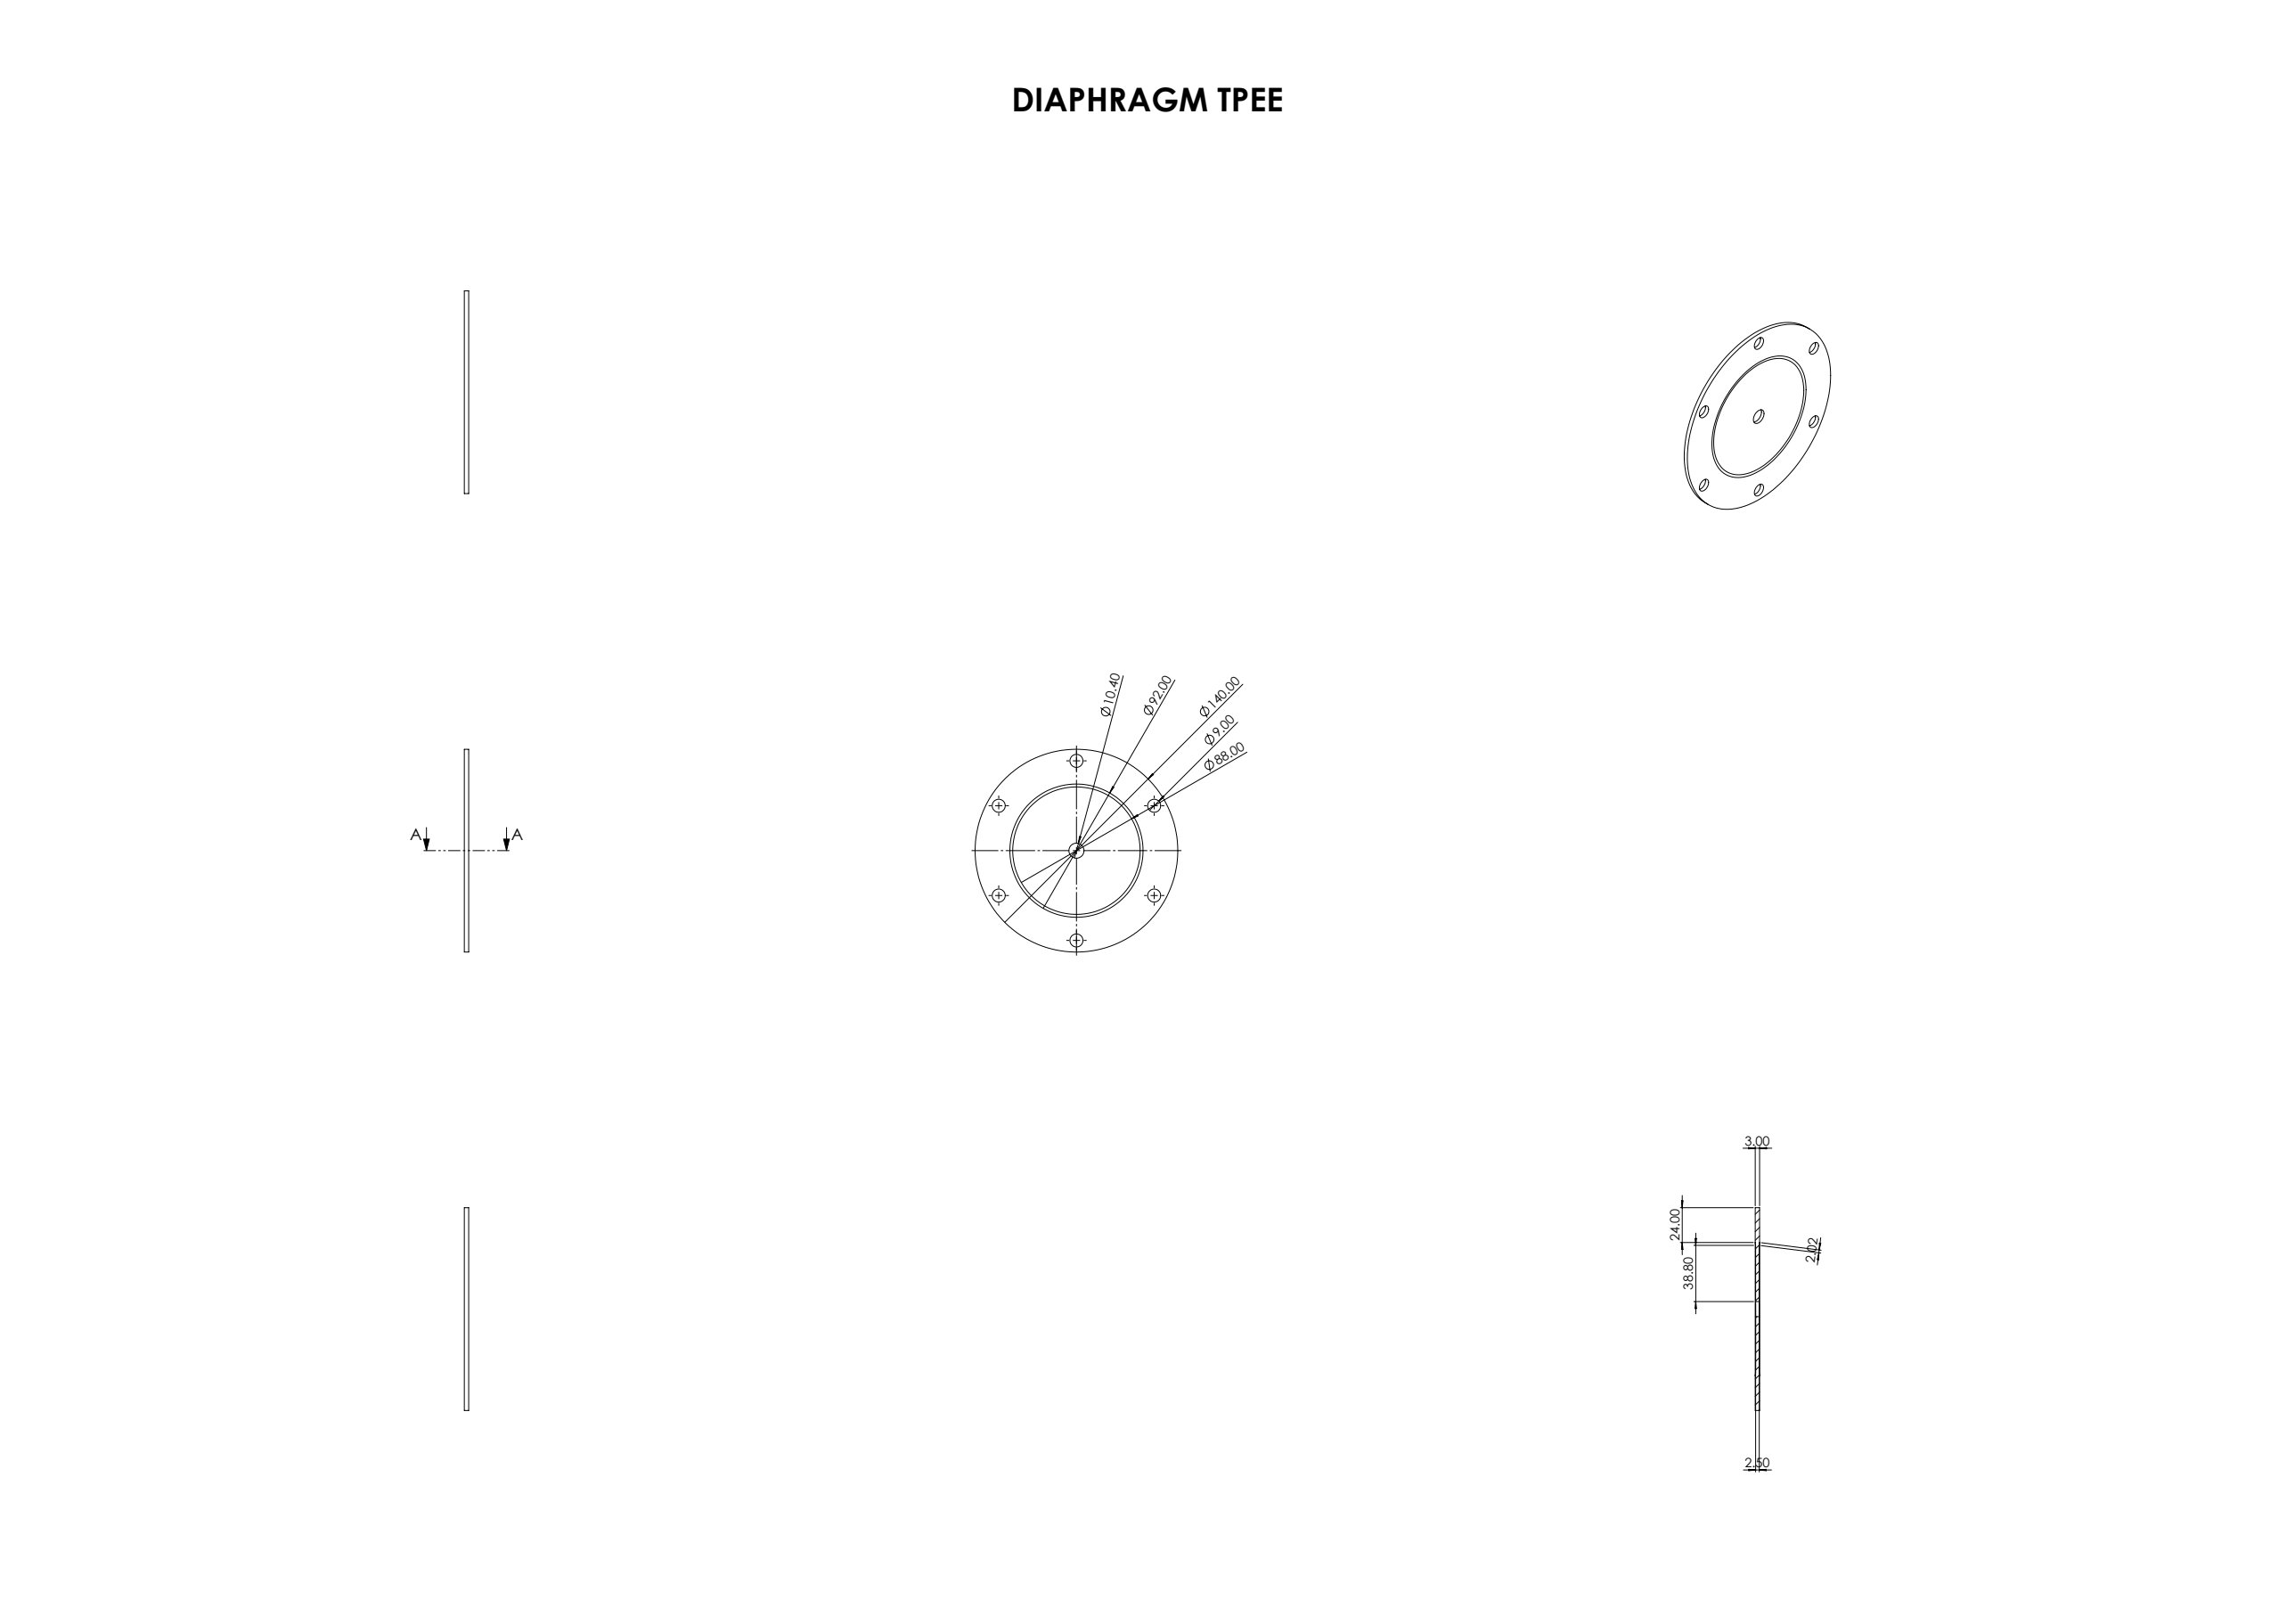
ISO-10303-21;
HEADER;
/* Generated by software containing ST-Developer
 * from STEP Tools, Inc. (www.steptools.com) 
 */

FILE_DESCRIPTION(
/* description */ (''),
/* implementation_level */ '2;1');

FILE_NAME(
/* name */ '05_Diaphragm_TPEE.step',
/* time_stamp */ '2026-10-26T06:13:19-07:00',
/* author */ (''),
/* organization */ (''),
/* preprocessor_version */ 'ST-DEVELOPER v20.2',
/* originating_system */ 'Autodesk Translation Framework v15.15.0.0',
/* authorisation */ '');

FILE_SCHEMA (('AUTOMOTIVE_DESIGN { 1 0 10303 214 3 1 1 }','TECHNICAL_DATA_PACKAGING'));
ENDSEC;

DATA;
#10=MECHANICAL_DESIGN_GEOMETRIC_PRESENTATION_REPRESENTATION('',(#301),#56639);
#261=SHAPE_REPRESENTATION_RELATIONSHIP('SRR','None',#56749,#281);
#281=ADVANCED_BREP_SHAPE_REPRESENTATION('',(#321),#56623);
#301=STYLED_ITEM('',(#56901),#321);
#321=MANIFOLD_SOLID_BREP('Body1',#16953);
#490=FACE_BOUND('',#3058,.T.);
#491=FACE_BOUND('',#3061,.T.);
#492=FACE_BOUND('',#3062,.T.);
#493=FACE_BOUND('',#3063,.T.);
#494=FACE_BOUND('',#3064,.T.);
#495=FACE_BOUND('',#3065,.T.);
#496=FACE_BOUND('',#3066,.T.);
#497=FACE_BOUND('',#3067,.T.);
#498=FACE_BOUND('',#3070,.T.);
#499=FACE_BOUND('',#3071,.T.);
#500=FACE_BOUND('',#3072,.T.);
#501=FACE_BOUND('',#3073,.T.);
#502=FACE_BOUND('',#3074,.T.);
#503=FACE_BOUND('',#3075,.T.);
#504=FACE_BOUND('',#3076,.T.);
#505=FACE_BOUND('',#3079,.T.);
#587=CONICAL_SURFACE('',#17639,45.,1.44644133224813);
#588=CONICAL_SURFACE('',#17647,45.,1.44644133224814);
#888=CIRCLE('',#17617,4.5);
#889=CIRCLE('',#17618,4.5);
#890=CIRCLE('',#17620,4.5);
#891=CIRCLE('',#17621,4.5);
#892=CIRCLE('',#17623,4.5);
#893=CIRCLE('',#17624,4.5);
#894=CIRCLE('',#17626,4.5);
#895=CIRCLE('',#17627,4.5);
#896=CIRCLE('',#17629,4.5);
#897=CIRCLE('',#17630,4.5);
#898=CIRCLE('',#17632,4.5);
#899=CIRCLE('',#17633,4.5);
#900=CIRCLE('',#17635,5.2);
#901=CIRCLE('',#17636,5.2);
#902=CIRCLE('',#17638,44.);
#903=CIRCLE('',#17640,46.);
#904=CIRCLE('',#17642,70.);
#905=CIRCLE('',#17644,70.);
#906=CIRCLE('',#17646,46.);
#907=CIRCLE('',#17648,44.);
#1309=CYLINDRICAL_SURFACE('',#17616,4.5);
#1310=CYLINDRICAL_SURFACE('',#17619,4.5);
#1311=CYLINDRICAL_SURFACE('',#17622,4.5);
#1312=CYLINDRICAL_SURFACE('',#17625,4.5);
#1313=CYLINDRICAL_SURFACE('',#17628,4.5);
#1314=CYLINDRICAL_SURFACE('',#17631,4.5);
#1315=CYLINDRICAL_SURFACE('',#17634,5.2);
#1316=CYLINDRICAL_SURFACE('',#17643,70.);
#2001=FACE_OUTER_BOUND('',#3050,.T.);
#2002=FACE_OUTER_BOUND('',#3051,.T.);
#2003=FACE_OUTER_BOUND('',#3052,.T.);
#2004=FACE_OUTER_BOUND('',#3053,.T.);
#2005=FACE_OUTER_BOUND('',#3054,.T.);
#2006=FACE_OUTER_BOUND('',#3055,.T.);
#2007=FACE_OUTER_BOUND('',#3056,.T.);
#2008=FACE_OUTER_BOUND('',#3057,.T.);
#2009=FACE_OUTER_BOUND('',#3059,.T.);
#2010=FACE_OUTER_BOUND('',#3060,.T.);
#2011=FACE_OUTER_BOUND('',#3068,.T.);
#2012=FACE_OUTER_BOUND('',#3069,.T.);
#2013=FACE_OUTER_BOUND('',#3077,.T.);
#2014=FACE_OUTER_BOUND('',#3078,.T.);
#3050=EDGE_LOOP('',(#11732,#11733,#11734,#11735));
#3051=EDGE_LOOP('',(#11736,#11737,#11738,#11739));
#3052=EDGE_LOOP('',(#11740,#11741,#11742,#11743));
#3053=EDGE_LOOP('',(#11744,#11745,#11746,#11747));
#3054=EDGE_LOOP('',(#11748,#11749,#11750,#11751));
#3055=EDGE_LOOP('',(#11752,#11753,#11754,#11755));
#3056=EDGE_LOOP('',(#11756,#11757,#11758,#11759));
#3057=EDGE_LOOP('',(#11760));
#3058=EDGE_LOOP('',(#11761));
#3059=EDGE_LOOP('',(#11762,#11763,#11764,#11765));
#3060=EDGE_LOOP('',(#11766));
#3061=EDGE_LOOP('',(#11767));
#3062=EDGE_LOOP('',(#11768));
#3063=EDGE_LOOP('',(#11769));
#3064=EDGE_LOOP('',(#11770));
#3065=EDGE_LOOP('',(#11771));
#3066=EDGE_LOOP('',(#11772));
#3067=EDGE_LOOP('',(#11773));
#3068=EDGE_LOOP('',(#11774,#11775,#11776,#11777));
#3069=EDGE_LOOP('',(#11778));
#3070=EDGE_LOOP('',(#11779));
#3071=EDGE_LOOP('',(#11780));
#3072=EDGE_LOOP('',(#11781));
#3073=EDGE_LOOP('',(#11782));
#3074=EDGE_LOOP('',(#11783));
#3075=EDGE_LOOP('',(#11784));
#3076=EDGE_LOOP('',(#11785));
#3077=EDGE_LOOP('',(#11786,#11787,#11788,#11789));
#3078=EDGE_LOOP('',(#11790));
#3079=EDGE_LOOP('',(#11791));
#4083=LINE('',#24999,#5037);
#4084=LINE('',#25005,#5038);
#4085=LINE('',#25011,#5039);
#4086=LINE('',#25017,#5040);
#4087=LINE('',#25023,#5041);
#4088=LINE('',#25029,#5042);
#4089=LINE('',#25035,#5043);
#4090=LINE('',#25042,#5044);
#4091=LINE('',#25050,#5045);
#4092=LINE('',#25056,#5046);
#5037=VECTOR('',#19827,4.5);
#5038=VECTOR('',#19834,4.5);
#5039=VECTOR('',#19841,4.5);
#5040=VECTOR('',#19848,4.5);
#5041=VECTOR('',#19855,4.5);
#5042=VECTOR('',#19862,4.5);
#5043=VECTOR('',#19869,5.2);
#5044=VECTOR('',#19878,45.);
#5045=VECTOR('',#19889,70.);
#5046=VECTOR('',#19896,45.);
#7019=VERTEX_POINT('',#24996);
#7020=VERTEX_POINT('',#24998);
#7021=VERTEX_POINT('',#25002);
#7022=VERTEX_POINT('',#25004);
#7023=VERTEX_POINT('',#25008);
#7024=VERTEX_POINT('',#25010);
#7025=VERTEX_POINT('',#25014);
#7026=VERTEX_POINT('',#25016);
#7027=VERTEX_POINT('',#25020);
#7028=VERTEX_POINT('',#25022);
#7029=VERTEX_POINT('',#25026);
#7030=VERTEX_POINT('',#25028);
#7031=VERTEX_POINT('',#25032);
#7032=VERTEX_POINT('',#25034);
#7033=VERTEX_POINT('',#25038);
#7034=VERTEX_POINT('',#25041);
#7035=VERTEX_POINT('',#25045);
#7036=VERTEX_POINT('',#25048);
#7037=VERTEX_POINT('',#25052);
#7038=VERTEX_POINT('',#25055);
#8773=EDGE_CURVE('',#7019,#7019,#888,.T.);
#8774=EDGE_CURVE('',#7019,#7020,#4083,.T.);
#8775=EDGE_CURVE('',#7020,#7020,#889,.T.);
#8776=EDGE_CURVE('',#7021,#7021,#890,.T.);
#8777=EDGE_CURVE('',#7021,#7022,#4084,.T.);
#8778=EDGE_CURVE('',#7022,#7022,#891,.T.);
#8779=EDGE_CURVE('',#7023,#7023,#892,.T.);
#8780=EDGE_CURVE('',#7023,#7024,#4085,.T.);
#8781=EDGE_CURVE('',#7024,#7024,#893,.T.);
#8782=EDGE_CURVE('',#7025,#7025,#894,.T.);
#8783=EDGE_CURVE('',#7025,#7026,#4086,.T.);
#8784=EDGE_CURVE('',#7026,#7026,#895,.T.);
#8785=EDGE_CURVE('',#7027,#7027,#896,.T.);
#8786=EDGE_CURVE('',#7027,#7028,#4087,.T.);
#8787=EDGE_CURVE('',#7028,#7028,#897,.T.);
#8788=EDGE_CURVE('',#7029,#7029,#898,.T.);
#8789=EDGE_CURVE('',#7029,#7030,#4088,.T.);
#8790=EDGE_CURVE('',#7030,#7030,#899,.T.);
#8791=EDGE_CURVE('',#7031,#7031,#900,.T.);
#8792=EDGE_CURVE('',#7031,#7032,#4089,.T.);
#8793=EDGE_CURVE('',#7032,#7032,#901,.T.);
#8794=EDGE_CURVE('',#7033,#7033,#902,.T.);
#8795=EDGE_CURVE('',#7033,#7034,#4090,.T.);
#8796=EDGE_CURVE('',#7034,#7034,#903,.T.);
#8797=EDGE_CURVE('',#7035,#7035,#904,.T.);
#8798=EDGE_CURVE('',#7036,#7036,#905,.T.);
#8799=EDGE_CURVE('',#7036,#7035,#4091,.T.);
#8800=EDGE_CURVE('',#7037,#7037,#906,.T.);
#8801=EDGE_CURVE('',#7037,#7038,#4092,.T.);
#8802=EDGE_CURVE('',#7038,#7038,#907,.T.);
#11732=ORIENTED_EDGE('',*,*,#8773,.F.);
#11733=ORIENTED_EDGE('',*,*,#8774,.T.);
#11734=ORIENTED_EDGE('',*,*,#8775,.F.);
#11735=ORIENTED_EDGE('',*,*,#8774,.F.);
#11736=ORIENTED_EDGE('',*,*,#8776,.F.);
#11737=ORIENTED_EDGE('',*,*,#8777,.T.);
#11738=ORIENTED_EDGE('',*,*,#8778,.F.);
#11739=ORIENTED_EDGE('',*,*,#8777,.F.);
#11740=ORIENTED_EDGE('',*,*,#8779,.F.);
#11741=ORIENTED_EDGE('',*,*,#8780,.T.);
#11742=ORIENTED_EDGE('',*,*,#8781,.F.);
#11743=ORIENTED_EDGE('',*,*,#8780,.F.);
#11744=ORIENTED_EDGE('',*,*,#8782,.F.);
#11745=ORIENTED_EDGE('',*,*,#8783,.T.);
#11746=ORIENTED_EDGE('',*,*,#8784,.F.);
#11747=ORIENTED_EDGE('',*,*,#8783,.F.);
#11748=ORIENTED_EDGE('',*,*,#8785,.F.);
#11749=ORIENTED_EDGE('',*,*,#8786,.T.);
#11750=ORIENTED_EDGE('',*,*,#8787,.F.);
#11751=ORIENTED_EDGE('',*,*,#8786,.F.);
#11752=ORIENTED_EDGE('',*,*,#8788,.F.);
#11753=ORIENTED_EDGE('',*,*,#8789,.T.);
#11754=ORIENTED_EDGE('',*,*,#8790,.F.);
#11755=ORIENTED_EDGE('',*,*,#8789,.F.);
#11756=ORIENTED_EDGE('',*,*,#8791,.T.);
#11757=ORIENTED_EDGE('',*,*,#8792,.T.);
#11758=ORIENTED_EDGE('',*,*,#8793,.F.);
#11759=ORIENTED_EDGE('',*,*,#8792,.F.);
#11760=ORIENTED_EDGE('',*,*,#8794,.F.);
#11761=ORIENTED_EDGE('',*,*,#8793,.T.);
#11762=ORIENTED_EDGE('',*,*,#8794,.T.);
#11763=ORIENTED_EDGE('',*,*,#8795,.T.);
#11764=ORIENTED_EDGE('',*,*,#8796,.F.);
#11765=ORIENTED_EDGE('',*,*,#8795,.F.);
#11766=ORIENTED_EDGE('',*,*,#8797,.F.);
#11767=ORIENTED_EDGE('',*,*,#8796,.T.);
#11768=ORIENTED_EDGE('',*,*,#8788,.T.);
#11769=ORIENTED_EDGE('',*,*,#8785,.T.);
#11770=ORIENTED_EDGE('',*,*,#8782,.T.);
#11771=ORIENTED_EDGE('',*,*,#8779,.T.);
#11772=ORIENTED_EDGE('',*,*,#8776,.T.);
#11773=ORIENTED_EDGE('',*,*,#8773,.T.);
#11774=ORIENTED_EDGE('',*,*,#8798,.F.);
#11775=ORIENTED_EDGE('',*,*,#8799,.T.);
#11776=ORIENTED_EDGE('',*,*,#8797,.T.);
#11777=ORIENTED_EDGE('',*,*,#8799,.F.);
#11778=ORIENTED_EDGE('',*,*,#8798,.T.);
#11779=ORIENTED_EDGE('',*,*,#8800,.F.);
#11780=ORIENTED_EDGE('',*,*,#8790,.T.);
#11781=ORIENTED_EDGE('',*,*,#8787,.T.);
#11782=ORIENTED_EDGE('',*,*,#8784,.T.);
#11783=ORIENTED_EDGE('',*,*,#8781,.T.);
#11784=ORIENTED_EDGE('',*,*,#8778,.T.);
#11785=ORIENTED_EDGE('',*,*,#8775,.T.);
#11786=ORIENTED_EDGE('',*,*,#8800,.T.);
#11787=ORIENTED_EDGE('',*,*,#8801,.T.);
#11788=ORIENTED_EDGE('',*,*,#8802,.F.);
#11789=ORIENTED_EDGE('',*,*,#8801,.F.);
#11790=ORIENTED_EDGE('',*,*,#8802,.T.);
#11791=ORIENTED_EDGE('',*,*,#8791,.F.);
#15775=PLANE('',#17637);
#15776=PLANE('',#17641);
#15777=PLANE('',#17645);
#15778=PLANE('',#17649);
#16172=ADVANCED_FACE('',(#2001),#1309,.F.);
#16173=ADVANCED_FACE('',(#2002),#1310,.F.);
#16174=ADVANCED_FACE('',(#2003),#1311,.F.);
#16175=ADVANCED_FACE('',(#2004),#1312,.F.);
#16176=ADVANCED_FACE('',(#2005),#1313,.F.);
#16177=ADVANCED_FACE('',(#2006),#1314,.F.);
#16178=ADVANCED_FACE('',(#2007),#1315,.F.);
#16179=ADVANCED_FACE('',(#2008,#490),#15775,.T.);
#16180=ADVANCED_FACE('',(#2009),#587,.F.);
#16181=ADVANCED_FACE('',(#2010,#491,#492,#493,#494,#495,#496,#497),#15776,
 .T.);
#16182=ADVANCED_FACE('',(#2011),#1316,.T.);
#16183=ADVANCED_FACE('',(#2012,#498,#499,#500,#501,#502,#503,#504),#15777,
 .T.);
#16184=ADVANCED_FACE('',(#2013),#588,.F.);
#16185=ADVANCED_FACE('',(#2014,#505),#15778,.T.);
#16953=CLOSED_SHELL('',(#16172,#16173,#16174,#16175,#16176,#16177,#16178,
#16179,#16180,#16181,#16182,#16183,#16184,#16185));
#17615=AXIS2_PLACEMENT_3D('',#24994,#19821,#19822);
#17616=AXIS2_PLACEMENT_3D('',#24995,#19823,#19824);
#17617=AXIS2_PLACEMENT_3D('',#24997,#19825,#19826);
#17618=AXIS2_PLACEMENT_3D('',#25000,#19828,#19829);
#17619=AXIS2_PLACEMENT_3D('',#25001,#19830,#19831);
#17620=AXIS2_PLACEMENT_3D('',#25003,#19832,#19833);
#17621=AXIS2_PLACEMENT_3D('',#25006,#19835,#19836);
#17622=AXIS2_PLACEMENT_3D('',#25007,#19837,#19838);
#17623=AXIS2_PLACEMENT_3D('',#25009,#19839,#19840);
#17624=AXIS2_PLACEMENT_3D('',#25012,#19842,#19843);
#17625=AXIS2_PLACEMENT_3D('',#25013,#19844,#19845);
#17626=AXIS2_PLACEMENT_3D('',#25015,#19846,#19847);
#17627=AXIS2_PLACEMENT_3D('',#25018,#19849,#19850);
#17628=AXIS2_PLACEMENT_3D('',#25019,#19851,#19852);
#17629=AXIS2_PLACEMENT_3D('',#25021,#19853,#19854);
#17630=AXIS2_PLACEMENT_3D('',#25024,#19856,#19857);
#17631=AXIS2_PLACEMENT_3D('',#25025,#19858,#19859);
#17632=AXIS2_PLACEMENT_3D('',#25027,#19860,#19861);
#17633=AXIS2_PLACEMENT_3D('',#25030,#19863,#19864);
#17634=AXIS2_PLACEMENT_3D('',#25031,#19865,#19866);
#17635=AXIS2_PLACEMENT_3D('',#25033,#19867,#19868);
#17636=AXIS2_PLACEMENT_3D('',#25036,#19870,#19871);
#17637=AXIS2_PLACEMENT_3D('',#25037,#19872,#19873);
#17638=AXIS2_PLACEMENT_3D('',#25039,#19874,#19875);
#17639=AXIS2_PLACEMENT_3D('',#25040,#19876,#19877);
#17640=AXIS2_PLACEMENT_3D('',#25043,#19879,#19880);
#17641=AXIS2_PLACEMENT_3D('',#25044,#19881,#19882);
#17642=AXIS2_PLACEMENT_3D('',#25046,#19883,#19884);
#17643=AXIS2_PLACEMENT_3D('',#25047,#19885,#19886);
#17644=AXIS2_PLACEMENT_3D('',#25049,#19887,#19888);
#17645=AXIS2_PLACEMENT_3D('',#25051,#19890,#19891);
#17646=AXIS2_PLACEMENT_3D('',#25053,#19892,#19893);
#17647=AXIS2_PLACEMENT_3D('',#25054,#19894,#19895);
#17648=AXIS2_PLACEMENT_3D('',#25057,#19897,#19898);
#17649=AXIS2_PLACEMENT_3D('',#25058,#19899,#19900);
#19821=DIRECTION('axis',(0.,0.,1.));
#19822=DIRECTION('refdir',(1.,0.,0.));
#19823=DIRECTION('center_axis',(1.,0.,0.));
#19824=DIRECTION('ref_axis',(0.,0.,-1.));
#19825=DIRECTION('center_axis',(1.,0.,0.));
#19826=DIRECTION('ref_axis',(0.,0.,-1.));
#19827=DIRECTION('',(1.,0.,0.));
#19828=DIRECTION('center_axis',(-1.,0.,0.));
#19829=DIRECTION('ref_axis',(0.,0.,-1.));
#19830=DIRECTION('center_axis',(1.,0.,0.));
#19831=DIRECTION('ref_axis',(0.,0.,-1.));
#19832=DIRECTION('center_axis',(1.,0.,0.));
#19833=DIRECTION('ref_axis',(0.,0.,-1.));
#19834=DIRECTION('',(1.,0.,0.));
#19835=DIRECTION('center_axis',(-1.,0.,0.));
#19836=DIRECTION('ref_axis',(0.,0.,-1.));
#19837=DIRECTION('center_axis',(1.,0.,0.));
#19838=DIRECTION('ref_axis',(0.,0.,-1.));
#19839=DIRECTION('center_axis',(1.,0.,0.));
#19840=DIRECTION('ref_axis',(0.,0.,-1.));
#19841=DIRECTION('',(1.,0.,0.));
#19842=DIRECTION('center_axis',(-1.,0.,0.));
#19843=DIRECTION('ref_axis',(0.,0.,-1.));
#19844=DIRECTION('center_axis',(1.,0.,0.));
#19845=DIRECTION('ref_axis',(0.,0.,-1.));
#19846=DIRECTION('center_axis',(1.,0.,0.));
#19847=DIRECTION('ref_axis',(0.,0.,-1.));
#19848=DIRECTION('',(1.,0.,0.));
#19849=DIRECTION('center_axis',(-1.,0.,0.));
#19850=DIRECTION('ref_axis',(0.,0.,-1.));
#19851=DIRECTION('center_axis',(1.,0.,0.));
#19852=DIRECTION('ref_axis',(0.,0.,-1.));
#19853=DIRECTION('center_axis',(1.,0.,0.));
#19854=DIRECTION('ref_axis',(0.,0.,-1.));
#19855=DIRECTION('',(1.,0.,0.));
#19856=DIRECTION('center_axis',(-1.,0.,0.));
#19857=DIRECTION('ref_axis',(0.,0.,-1.));
#19858=DIRECTION('center_axis',(1.,0.,0.));
#19859=DIRECTION('ref_axis',(0.,0.,-1.));
#19860=DIRECTION('center_axis',(1.,0.,0.));
#19861=DIRECTION('ref_axis',(0.,0.,-1.));
#19862=DIRECTION('',(1.,0.,0.));
#19863=DIRECTION('center_axis',(-1.,0.,0.));
#19864=DIRECTION('ref_axis',(0.,0.,-1.));
#19865=DIRECTION('center_axis',(1.,0.,0.));
#19866=DIRECTION('ref_axis',(0.,1.,0.));
#19867=DIRECTION('center_axis',(1.,0.,0.));
#19868=DIRECTION('ref_axis',(0.,0.,-1.));
#19869=DIRECTION('',(-1.,0.,0.));
#19870=DIRECTION('center_axis',(1.,0.,0.));
#19871=DIRECTION('ref_axis',(0.,0.,-1.));
#19872=DIRECTION('center_axis',(-1.,0.,0.));
#19873=DIRECTION('ref_axis',(0.,0.,1.));
#19874=DIRECTION('center_axis',(1.,0.,0.));
#19875=DIRECTION('ref_axis',(0.,0.,-1.));
#19876=DIRECTION('center_axis',(-1.,0.,0.));
#19877=DIRECTION('ref_axis',(0.,1.,0.));
#19878=DIRECTION('',(-0.124034734589211,-0.992277876713667,-1.21518992558212E-16));
#19879=DIRECTION('center_axis',(1.,0.,0.));
#19880=DIRECTION('ref_axis',(0.,0.,-1.));
#19881=DIRECTION('center_axis',(-1.,0.,0.));
#19882=DIRECTION('ref_axis',(0.,0.,1.));
#19883=DIRECTION('center_axis',(1.,0.,0.));
#19884=DIRECTION('ref_axis',(0.,0.,-1.));
#19885=DIRECTION('center_axis',(1.,0.,0.));
#19886=DIRECTION('ref_axis',(0.,1.,0.));
#19887=DIRECTION('center_axis',(1.,0.,0.));
#19888=DIRECTION('ref_axis',(0.,0.,-1.));
#19889=DIRECTION('',(-1.,0.,0.));
#19890=DIRECTION('center_axis',(1.,0.,0.));
#19891=DIRECTION('ref_axis',(0.,0.,-1.));
#19892=DIRECTION('center_axis',(1.,0.,0.));
#19893=DIRECTION('ref_axis',(0.,0.,-1.));
#19894=DIRECTION('center_axis',(1.,0.,0.));
#19895=DIRECTION('ref_axis',(0.,1.,0.));
#19896=DIRECTION('',(-0.124034734589208,0.992277876713668,1.21518992558212E-16));
#19897=DIRECTION('center_axis',(1.,0.,0.));
#19898=DIRECTION('ref_axis',(0.,0.,-1.));
#19899=DIRECTION('center_axis',(1.,0.,0.));
#19900=DIRECTION('ref_axis',(0.,0.,-1.));
#24994=CARTESIAN_POINT('',(0.,0.,0.));
#24995=CARTESIAN_POINT('Origin',(35.4,-31.,-53.6935750346352));
#24996=CARTESIAN_POINT('',(35.5,-31.,-49.1935750346352));
#24997=CARTESIAN_POINT('Origin',(35.5,-31.,-53.6935750346352));
#24998=CARTESIAN_POINT('',(38.5,-31.,-49.1935750346352));
#24999=CARTESIAN_POINT('',(35.4,-31.,-49.1935750346352));
#25000=CARTESIAN_POINT('Origin',(38.5,-31.,-53.6935750346352));
#25001=CARTESIAN_POINT('Origin',(35.4,62.,0.));
#25002=CARTESIAN_POINT('',(35.5,62.,4.5));
#25003=CARTESIAN_POINT('Origin',(35.5,62.,0.));
#25004=CARTESIAN_POINT('',(38.5,62.,4.5));
#25005=CARTESIAN_POINT('',(35.4,62.,4.5));
#25006=CARTESIAN_POINT('Origin',(38.5,62.,0.));
#25007=CARTESIAN_POINT('Origin',(35.4,31.,53.6935750346352));
#25008=CARTESIAN_POINT('',(35.5,31.,58.1935750346352));
#25009=CARTESIAN_POINT('Origin',(35.5,31.,53.6935750346352));
#25010=CARTESIAN_POINT('',(38.5,31.,58.1935750346352));
#25011=CARTESIAN_POINT('',(35.4,31.,58.1935750346352));
#25012=CARTESIAN_POINT('Origin',(38.5,31.,53.6935750346352));
#25013=CARTESIAN_POINT('Origin',(35.4,-31.,53.6935750346352));
#25014=CARTESIAN_POINT('',(35.5,-31.,58.1935750346352));
#25015=CARTESIAN_POINT('Origin',(35.5,-31.,53.6935750346352));
#25016=CARTESIAN_POINT('',(38.5,-31.,58.1935750346352));
#25017=CARTESIAN_POINT('',(35.4,-31.,58.1935750346352));
#25018=CARTESIAN_POINT('Origin',(38.5,-31.,53.6935750346352));
#25019=CARTESIAN_POINT('Origin',(35.4,-62.,7.59281015471359E-15));
#25020=CARTESIAN_POINT('',(35.5,-62.,4.50000000000001));
#25021=CARTESIAN_POINT('Origin',(35.5,-62.,7.59281015471359E-15));
#25022=CARTESIAN_POINT('',(38.5,-62.,4.50000000000001));
#25023=CARTESIAN_POINT('',(35.4,-62.,4.50000000000001));
#25024=CARTESIAN_POINT('Origin',(38.5,-62.,7.59281015471359E-15));
#25025=CARTESIAN_POINT('Origin',(35.4,31.,-53.6935750346352));
#25026=CARTESIAN_POINT('',(35.5,31.,-49.1935750346352));
#25027=CARTESIAN_POINT('Origin',(35.5,31.,-53.6935750346352));
#25028=CARTESIAN_POINT('',(38.5,31.,-49.1935750346352));
#25029=CARTESIAN_POINT('',(35.4,31.,-49.1935750346352));
#25030=CARTESIAN_POINT('Origin',(38.5,31.,-53.6935750346352));
#25031=CARTESIAN_POINT('Origin',(37.,0.,0.));
#25032=CARTESIAN_POINT('',(38.25,-5.2,-6.36816335556624E-16));
#25033=CARTESIAN_POINT('Origin',(38.25,0.,0.));
#25034=CARTESIAN_POINT('',(35.75,-5.2,-6.36816335556624E-16));
#25035=CARTESIAN_POINT('',(37.,-5.2,-6.36816335556624E-16));
#25036=CARTESIAN_POINT('Origin',(35.75,0.,0.));
#25037=CARTESIAN_POINT('Origin',(35.75,44.,0.));
#25038=CARTESIAN_POINT('',(35.75,-44.,-5.38844591624835E-15));
#25039=CARTESIAN_POINT('Origin',(35.75,0.,0.));
#25040=CARTESIAN_POINT('Origin',(35.625,0.,0.));
#25041=CARTESIAN_POINT('',(35.5,-46.,-5.63337527607782E-15));
#25042=CARTESIAN_POINT('',(35.625,-45.,-5.51091059616309E-15));
#25043=CARTESIAN_POINT('Origin',(35.5,0.,0.));
#25044=CARTESIAN_POINT('Origin',(35.5,70.,0.));
#25045=CARTESIAN_POINT('',(35.5,-70.,-8.57252759403147E-15));
#25046=CARTESIAN_POINT('Origin',(35.5,0.,0.));
#25047=CARTESIAN_POINT('Origin',(37.,0.,0.));
#25048=CARTESIAN_POINT('',(38.5,-70.,-8.57252759403147E-15));
#25049=CARTESIAN_POINT('Origin',(38.5,0.,0.));
#25050=CARTESIAN_POINT('',(37.,-70.,-8.57252759403147E-15));
#25051=CARTESIAN_POINT('Origin',(38.5,46.,0.));
#25052=CARTESIAN_POINT('',(38.5,-46.,-5.63337527607782E-15));
#25053=CARTESIAN_POINT('Origin',(38.5,0.,0.));
#25054=CARTESIAN_POINT('Origin',(38.375,0.,0.));
#25055=CARTESIAN_POINT('',(38.25,-44.,-5.38844591624835E-15));
#25056=CARTESIAN_POINT('',(38.375,-45.,-5.51091059616309E-15));
#25057=CARTESIAN_POINT('Origin',(38.25,0.,0.));
#25058=CARTESIAN_POINT('Origin',(38.25,5.2,0.));
#56601=UNCERTAINTY_MEASURE_WITH_UNIT(LENGTH_MEASURE(0.01),#56640,
'DISTANCE_ACCURACY_VALUE',
'Maximum model space distance between geometric entities at asserted c
onnectivities');
#56617=UNCERTAINTY_MEASURE_WITH_UNIT(LENGTH_MEASURE(0.01),#56640,
'DISTANCE_ACCURACY_VALUE',
'Maximum model space distance between geometric entities at asserted c
onnectivities');
#56623=(
GEOMETRIC_REPRESENTATION_CONTEXT(3)
GLOBAL_UNCERTAINTY_ASSIGNED_CONTEXT((#56601))
GLOBAL_UNIT_ASSIGNED_CONTEXT((#56640,#56642,#56643))
REPRESENTATION_CONTEXT('','3D')
);
#56639=(
GEOMETRIC_REPRESENTATION_CONTEXT(3)
GLOBAL_UNCERTAINTY_ASSIGNED_CONTEXT((#56617))
GLOBAL_UNIT_ASSIGNED_CONTEXT((#56640,#56642,#56643))
REPRESENTATION_CONTEXT('','3D')
);
#56640=(
LENGTH_UNIT()
NAMED_UNIT(*)
SI_UNIT(.MILLI.,.METRE.)
);
#56642=(
NAMED_UNIT(*)
PLANE_ANGLE_UNIT()
SI_UNIT($,.RADIAN.)
);
#56643=(
NAMED_UNIT(*)
SI_UNIT($,.STERADIAN.)
SOLID_ANGLE_UNIT()
);
#56649=SHAPE_DEFINITION_REPRESENTATION(#56670,#56749);
#56670=PRODUCT_DEFINITION_SHAPE('',$,#56771);
#56749=SHAPE_REPRESENTATION('',(#17615),#56623);
#56765=PRODUCT_DEFINITION_CONTEXT('part definition',#56830,'design');
#56771=PRODUCT_DEFINITION('2026-10-26-00-02-41-508','05_Diaphragm_TPEE',
#56792,#56765);
#56792=PRODUCT_DEFINITION_FORMATION('',$,#56837);
#56830=APPLICATION_CONTEXT(
'Core Data for Automotive Mechanical Design Process');
#56831=PRODUCT_CONTEXT('part definition',#56830,'mechanical');
#56837=PRODUCT('2026-10-26-00-02-41-508','05_Diaphragm_TPEE',$,(#56831));
#56895=COLOUR_RGB('Light Blue',0.38,0.62,0.78);
#56896=FILL_AREA_STYLE_COLOUR('',#56895);
#56897=FILL_AREA_STYLE('',(#56896));
#56898=SURFACE_STYLE_FILL_AREA(#56897);
#56899=SURFACE_SIDE_STYLE('',(#56898));
#56900=SURFACE_STYLE_USAGE(.BOTH.,#56899);
#56901=PRESENTATION_STYLE_ASSIGNMENT((#56900));
ENDSEC;
END-ISO-10303-21;
